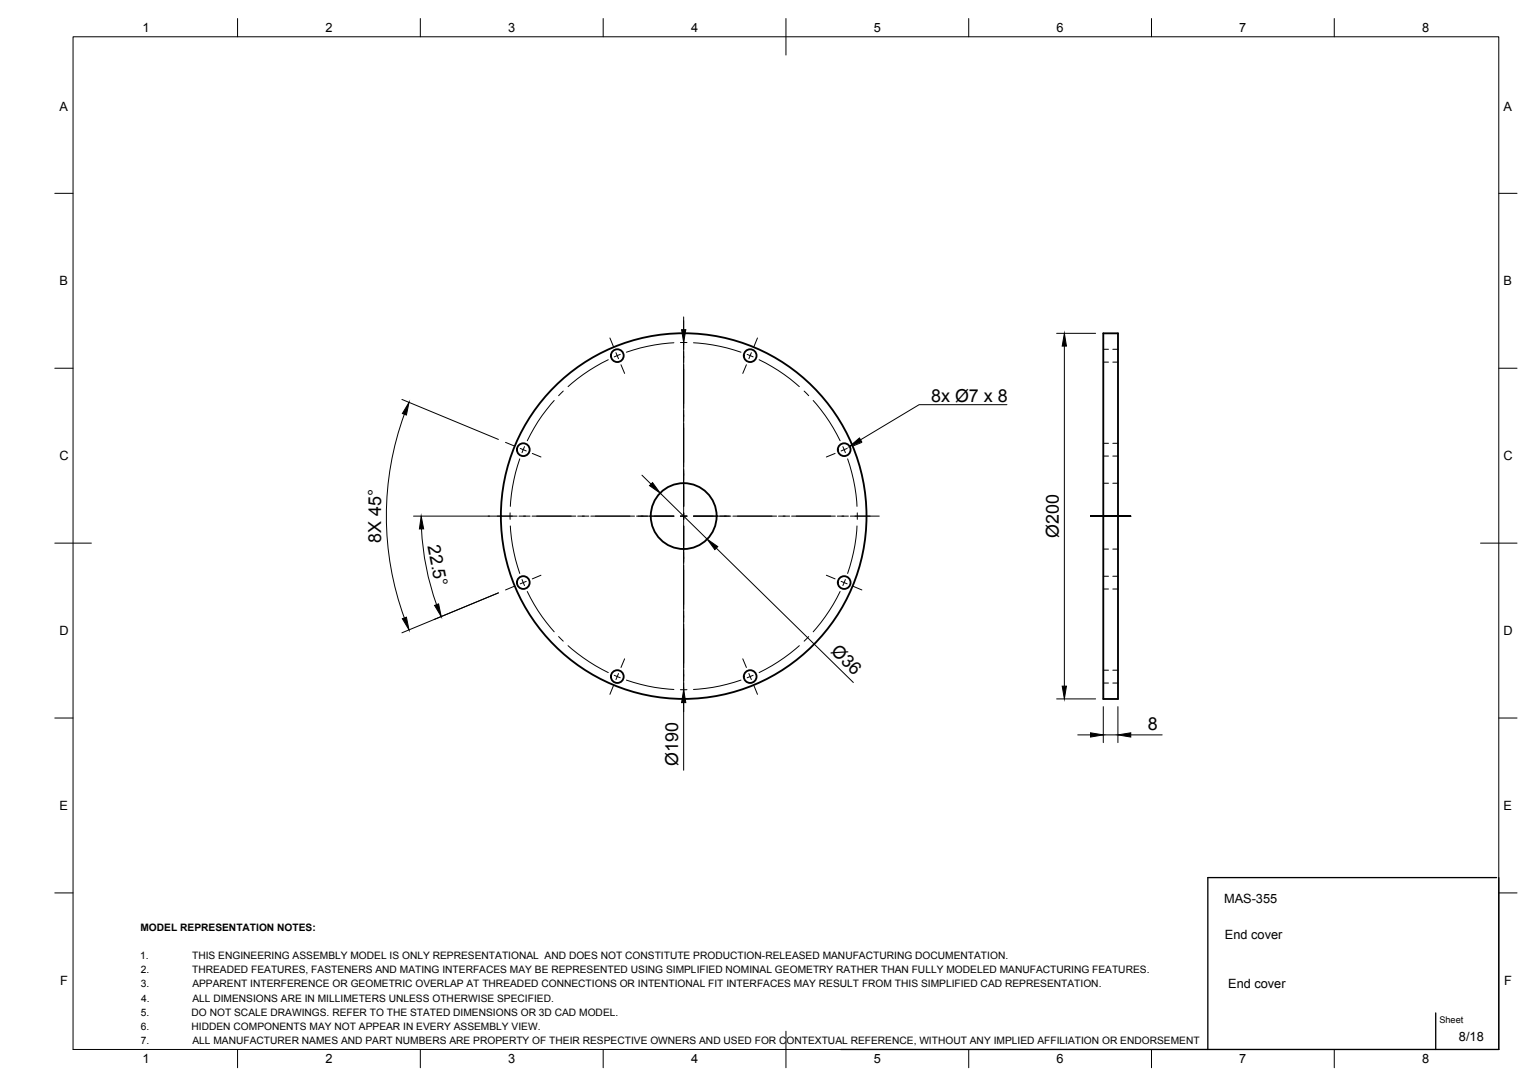
ISO-10303-21;
HEADER;
/* Generated by software containing ST-Developer
 * from STEP Tools, Inc. (www.steptools.com) 
 */

FILE_DESCRIPTION(
/* description */ ('Independent two-stage fixed-ring planetary gearbox,24/24/72 teeth,mod
ule2,20deg involutes,three planets per stage,4:1 x4:1=16:1. Native cut
-space/fillet/pattern tooth profiles derived from reusable gear blanks
; shared sun/planet/ring/carrier parts across both stages. Captured br
onze-journal input/carriers, headed retained planet pins, keyed inters
tage drive and modular keyed output interface. Native ideal gear links
; no torque, precision grade, production backlash/fits, lubrication, s
peed or life rating.'),
/* implementation_level */ '2;1');

FILE_NAME(
/* name */ 'End cover.step',
/* time_stamp */ '2026-11-08T19:10:00-08:00',
/* author */ (''),
/* organization */ (''),
/* preprocessor_version */ 'ST-DEVELOPER v20.2',
/* originating_system */ 'Autodesk Translation Framework v15.17.0.0',
/* authorisation */ '');

FILE_SCHEMA (('AUTOMOTIVE_DESIGN { 1 0 10303 214 3 1 1 }'));
ENDSEC;

DATA;
#10=MECHANICAL_DESIGN_GEOMETRIC_PRESENTATION_REPRESENTATION('',(#1165),#259224);
#1125=SHAPE_REPRESENTATION_RELATIONSHIP('SRR','None',#259372,#1145);
#1145=ADVANCED_BREP_SHAPE_REPRESENTATION('',(#1185),#259206);
#1165=STYLED_ITEM('',(#259481),#1185);
#1185=MANIFOLD_SOLID_BREP('Body1',#25152);
#1247=FACE_BOUND('',#3425,.T.);
#1248=FACE_BOUND('',#3426,.T.);
#1249=FACE_BOUND('',#3427,.T.);
#1250=FACE_BOUND('',#3428,.T.);
#1251=FACE_BOUND('',#3429,.T.);
#1252=FACE_BOUND('',#3430,.T.);
#1253=FACE_BOUND('',#3431,.T.);
#1254=FACE_BOUND('',#3432,.T.);
#1255=FACE_BOUND('',#3433,.T.);
#1256=FACE_BOUND('',#3435,.T.);
#1257=FACE_BOUND('',#3436,.T.);
#1258=FACE_BOUND('',#3437,.T.);
#1259=FACE_BOUND('',#3438,.T.);
#1260=FACE_BOUND('',#3439,.T.);
#1261=FACE_BOUND('',#3440,.T.);
#1262=FACE_BOUND('',#3441,.T.);
#1263=FACE_BOUND('',#3442,.T.);
#1264=FACE_BOUND('',#3443,.T.);
#1507=PLANE('',#25809);
#1508=PLANE('',#25810);
#2024=FACE_OUTER_BOUND('',#3414,.T.);
#2025=FACE_OUTER_BOUND('',#3415,.T.);
#2026=FACE_OUTER_BOUND('',#3416,.T.);
#2027=FACE_OUTER_BOUND('',#3417,.T.);
#2028=FACE_OUTER_BOUND('',#3418,.T.);
#2029=FACE_OUTER_BOUND('',#3419,.T.);
#2030=FACE_OUTER_BOUND('',#3420,.T.);
#2031=FACE_OUTER_BOUND('',#3421,.T.);
#2032=FACE_OUTER_BOUND('',#3422,.T.);
#2033=FACE_OUTER_BOUND('',#3423,.T.);
#2034=FACE_OUTER_BOUND('',#3424,.T.);
#2035=FACE_OUTER_BOUND('',#3434,.T.);
#3414=EDGE_LOOP('',(#17352,#17353,#17354,#17355));
#3415=EDGE_LOOP('',(#17356,#17357,#17358,#17359));
#3416=EDGE_LOOP('',(#17360,#17361,#17362,#17363));
#3417=EDGE_LOOP('',(#17364,#17365,#17366,#17367));
#3418=EDGE_LOOP('',(#17368,#17369,#17370,#17371));
#3419=EDGE_LOOP('',(#17372,#17373,#17374,#17375));
#3420=EDGE_LOOP('',(#17376,#17377,#17378,#17379));
#3421=EDGE_LOOP('',(#17380,#17381,#17382,#17383));
#3422=EDGE_LOOP('',(#17384,#17385,#17386,#17387));
#3423=EDGE_LOOP('',(#17388,#17389,#17390,#17391));
#3424=EDGE_LOOP('',(#17392));
#3425=EDGE_LOOP('',(#17393));
#3426=EDGE_LOOP('',(#17394));
#3427=EDGE_LOOP('',(#17395));
#3428=EDGE_LOOP('',(#17396));
#3429=EDGE_LOOP('',(#17397));
#3430=EDGE_LOOP('',(#17398));
#3431=EDGE_LOOP('',(#17399));
#3432=EDGE_LOOP('',(#17400));
#3433=EDGE_LOOP('',(#17401));
#3434=EDGE_LOOP('',(#17402));
#3435=EDGE_LOOP('',(#17403));
#3436=EDGE_LOOP('',(#17404));
#3437=EDGE_LOOP('',(#17405));
#3438=EDGE_LOOP('',(#17406));
#3439=EDGE_LOOP('',(#17407));
#3440=EDGE_LOOP('',(#17408));
#3441=EDGE_LOOP('',(#17409));
#3442=EDGE_LOOP('',(#17410));
#3443=EDGE_LOOP('',(#17411));
#4579=CIRCLE('',#25780,3.5);
#4580=CIRCLE('',#25781,3.5);
#4581=CIRCLE('',#25783,3.5);
#4582=CIRCLE('',#25784,3.5);
#4583=CIRCLE('',#25786,3.5);
#4584=CIRCLE('',#25787,3.5);
#4585=CIRCLE('',#25789,3.5);
#4586=CIRCLE('',#25790,3.5);
#4587=CIRCLE('',#25792,3.5);
#4588=CIRCLE('',#25793,3.5);
#4589=CIRCLE('',#25795,3.5);
#4590=CIRCLE('',#25796,3.5);
#4591=CIRCLE('',#25798,3.5);
#4592=CIRCLE('',#25799,3.5);
#4593=CIRCLE('',#25801,3.5);
#4594=CIRCLE('',#25802,3.5);
#4595=CIRCLE('',#25804,18.);
#4596=CIRCLE('',#25805,18.);
#4597=CIRCLE('',#25807,100.);
#4598=CIRCLE('',#25808,100.);
#6949=LINE('',#52233,#8134);
#6950=LINE('',#52239,#8135);
#6951=LINE('',#52245,#8136);
#6952=LINE('',#52251,#8137);
#6953=LINE('',#52257,#8138);
#6954=LINE('',#52263,#8139);
#6955=LINE('',#52269,#8140);
#6956=LINE('',#52275,#8141);
#6957=LINE('',#52281,#8142);
#6958=LINE('',#52287,#8143);
#8134=VECTOR('',#28396,3.5);
#8135=VECTOR('',#28403,3.5);
#8136=VECTOR('',#28410,3.5);
#8137=VECTOR('',#28417,3.5);
#8138=VECTOR('',#28424,3.5);
#8139=VECTOR('',#28431,3.5);
#8140=VECTOR('',#28438,3.5);
#8141=VECTOR('',#28445,3.5);
#8142=VECTOR('',#28452,18.);
#8143=VECTOR('',#28459,100.);
#9687=VERTEX_POINT('',#52230);
#9688=VERTEX_POINT('',#52232);
#9689=VERTEX_POINT('',#52236);
#9690=VERTEX_POINT('',#52238);
#9691=VERTEX_POINT('',#52242);
#9692=VERTEX_POINT('',#52244);
#9693=VERTEX_POINT('',#52248);
#9694=VERTEX_POINT('',#52250);
#9695=VERTEX_POINT('',#52254);
#9696=VERTEX_POINT('',#52256);
#9697=VERTEX_POINT('',#52260);
#9698=VERTEX_POINT('',#52262);
#9699=VERTEX_POINT('',#52266);
#9700=VERTEX_POINT('',#52268);
#9701=VERTEX_POINT('',#52272);
#9702=VERTEX_POINT('',#52274);
#9703=VERTEX_POINT('',#52278);
#9704=VERTEX_POINT('',#52280);
#9705=VERTEX_POINT('',#52284);
#9706=VERTEX_POINT('',#52286);
#12561=EDGE_CURVE('',#9687,#9687,#4579,.T.);
#12562=EDGE_CURVE('',#9687,#9688,#6949,.T.);
#12563=EDGE_CURVE('',#9688,#9688,#4580,.T.);
#12564=EDGE_CURVE('',#9689,#9689,#4581,.T.);
#12565=EDGE_CURVE('',#9689,#9690,#6950,.T.);
#12566=EDGE_CURVE('',#9690,#9690,#4582,.T.);
#12567=EDGE_CURVE('',#9691,#9691,#4583,.T.);
#12568=EDGE_CURVE('',#9691,#9692,#6951,.T.);
#12569=EDGE_CURVE('',#9692,#9692,#4584,.T.);
#12570=EDGE_CURVE('',#9693,#9693,#4585,.T.);
#12571=EDGE_CURVE('',#9693,#9694,#6952,.T.);
#12572=EDGE_CURVE('',#9694,#9694,#4586,.T.);
#12573=EDGE_CURVE('',#9695,#9695,#4587,.T.);
#12574=EDGE_CURVE('',#9695,#9696,#6953,.T.);
#12575=EDGE_CURVE('',#9696,#9696,#4588,.T.);
#12576=EDGE_CURVE('',#9697,#9697,#4589,.T.);
#12577=EDGE_CURVE('',#9697,#9698,#6954,.T.);
#12578=EDGE_CURVE('',#9698,#9698,#4590,.T.);
#12579=EDGE_CURVE('',#9699,#9699,#4591,.T.);
#12580=EDGE_CURVE('',#9699,#9700,#6955,.T.);
#12581=EDGE_CURVE('',#9700,#9700,#4592,.T.);
#12582=EDGE_CURVE('',#9701,#9701,#4593,.T.);
#12583=EDGE_CURVE('',#9701,#9702,#6956,.T.);
#12584=EDGE_CURVE('',#9702,#9702,#4594,.T.);
#12585=EDGE_CURVE('',#9703,#9703,#4595,.T.);
#12586=EDGE_CURVE('',#9703,#9704,#6957,.T.);
#12587=EDGE_CURVE('',#9704,#9704,#4596,.T.);
#12588=EDGE_CURVE('',#9705,#9705,#4597,.T.);
#12589=EDGE_CURVE('',#9705,#9706,#6958,.T.);
#12590=EDGE_CURVE('',#9706,#9706,#4598,.T.);
#17352=ORIENTED_EDGE('',*,*,#12561,.F.);
#17353=ORIENTED_EDGE('',*,*,#12562,.T.);
#17354=ORIENTED_EDGE('',*,*,#12563,.F.);
#17355=ORIENTED_EDGE('',*,*,#12562,.F.);
#17356=ORIENTED_EDGE('',*,*,#12564,.F.);
#17357=ORIENTED_EDGE('',*,*,#12565,.T.);
#17358=ORIENTED_EDGE('',*,*,#12566,.F.);
#17359=ORIENTED_EDGE('',*,*,#12565,.F.);
#17360=ORIENTED_EDGE('',*,*,#12567,.F.);
#17361=ORIENTED_EDGE('',*,*,#12568,.T.);
#17362=ORIENTED_EDGE('',*,*,#12569,.F.);
#17363=ORIENTED_EDGE('',*,*,#12568,.F.);
#17364=ORIENTED_EDGE('',*,*,#12570,.F.);
#17365=ORIENTED_EDGE('',*,*,#12571,.T.);
#17366=ORIENTED_EDGE('',*,*,#12572,.F.);
#17367=ORIENTED_EDGE('',*,*,#12571,.F.);
#17368=ORIENTED_EDGE('',*,*,#12573,.F.);
#17369=ORIENTED_EDGE('',*,*,#12574,.T.);
#17370=ORIENTED_EDGE('',*,*,#12575,.F.);
#17371=ORIENTED_EDGE('',*,*,#12574,.F.);
#17372=ORIENTED_EDGE('',*,*,#12576,.F.);
#17373=ORIENTED_EDGE('',*,*,#12577,.T.);
#17374=ORIENTED_EDGE('',*,*,#12578,.F.);
#17375=ORIENTED_EDGE('',*,*,#12577,.F.);
#17376=ORIENTED_EDGE('',*,*,#12579,.F.);
#17377=ORIENTED_EDGE('',*,*,#12580,.T.);
#17378=ORIENTED_EDGE('',*,*,#12581,.F.);
#17379=ORIENTED_EDGE('',*,*,#12580,.F.);
#17380=ORIENTED_EDGE('',*,*,#12582,.F.);
#17381=ORIENTED_EDGE('',*,*,#12583,.T.);
#17382=ORIENTED_EDGE('',*,*,#12584,.F.);
#17383=ORIENTED_EDGE('',*,*,#12583,.F.);
#17384=ORIENTED_EDGE('',*,*,#12585,.F.);
#17385=ORIENTED_EDGE('',*,*,#12586,.T.);
#17386=ORIENTED_EDGE('',*,*,#12587,.T.);
#17387=ORIENTED_EDGE('',*,*,#12586,.F.);
#17388=ORIENTED_EDGE('',*,*,#12588,.F.);
#17389=ORIENTED_EDGE('',*,*,#12589,.T.);
#17390=ORIENTED_EDGE('',*,*,#12590,.T.);
#17391=ORIENTED_EDGE('',*,*,#12589,.F.);
#17392=ORIENTED_EDGE('',*,*,#12588,.T.);
#17393=ORIENTED_EDGE('',*,*,#12585,.T.);
#17394=ORIENTED_EDGE('',*,*,#12582,.T.);
#17395=ORIENTED_EDGE('',*,*,#12579,.T.);
#17396=ORIENTED_EDGE('',*,*,#12576,.T.);
#17397=ORIENTED_EDGE('',*,*,#12573,.T.);
#17398=ORIENTED_EDGE('',*,*,#12570,.T.);
#17399=ORIENTED_EDGE('',*,*,#12567,.T.);
#17400=ORIENTED_EDGE('',*,*,#12564,.T.);
#17401=ORIENTED_EDGE('',*,*,#12561,.T.);
#17402=ORIENTED_EDGE('',*,*,#12590,.F.);
#17403=ORIENTED_EDGE('',*,*,#12587,.F.);
#17404=ORIENTED_EDGE('',*,*,#12584,.T.);
#17405=ORIENTED_EDGE('',*,*,#12581,.T.);
#17406=ORIENTED_EDGE('',*,*,#12578,.T.);
#17407=ORIENTED_EDGE('',*,*,#12575,.T.);
#17408=ORIENTED_EDGE('',*,*,#12572,.T.);
#17409=ORIENTED_EDGE('',*,*,#12569,.T.);
#17410=ORIENTED_EDGE('',*,*,#12566,.T.);
#17411=ORIENTED_EDGE('',*,*,#12563,.T.);
#23361=CYLINDRICAL_SURFACE('',#25779,3.5);
#23362=CYLINDRICAL_SURFACE('',#25782,3.5);
#23363=CYLINDRICAL_SURFACE('',#25785,3.5);
#23364=CYLINDRICAL_SURFACE('',#25788,3.5);
#23365=CYLINDRICAL_SURFACE('',#25791,3.5);
#23366=CYLINDRICAL_SURFACE('',#25794,3.5);
#23367=CYLINDRICAL_SURFACE('',#25797,3.5);
#23368=CYLINDRICAL_SURFACE('',#25800,3.5);
#23369=CYLINDRICAL_SURFACE('',#25803,18.);
#23370=CYLINDRICAL_SURFACE('',#25806,100.);
#24130=ADVANCED_FACE('',(#2024),#23361,.F.);
#24131=ADVANCED_FACE('',(#2025),#23362,.F.);
#24132=ADVANCED_FACE('',(#2026),#23363,.F.);
#24133=ADVANCED_FACE('',(#2027),#23364,.F.);
#24134=ADVANCED_FACE('',(#2028),#23365,.F.);
#24135=ADVANCED_FACE('',(#2029),#23366,.F.);
#24136=ADVANCED_FACE('',(#2030),#23367,.F.);
#24137=ADVANCED_FACE('',(#2031),#23368,.F.);
#24138=ADVANCED_FACE('',(#2032),#23369,.F.);
#24139=ADVANCED_FACE('',(#2033),#23370,.T.);
#24140=ADVANCED_FACE('',(#2034,#1247,#1248,#1249,#1250,#1251,#1252,#1253,
#1254,#1255),#1507,.T.);
#24141=ADVANCED_FACE('',(#2035,#1256,#1257,#1258,#1259,#1260,#1261,#1262,
#1263,#1264),#1508,.F.);
#25152=CLOSED_SHELL('',(#24130,#24131,#24132,#24133,#24134,#24135,#24136,
#24137,#24138,#24139,#24140,#24141));
#25778=AXIS2_PLACEMENT_3D('',#52228,#28390,#28391);
#25779=AXIS2_PLACEMENT_3D('',#52229,#28392,#28393);
#25780=AXIS2_PLACEMENT_3D('',#52231,#28394,#28395);
#25781=AXIS2_PLACEMENT_3D('',#52234,#28397,#28398);
#25782=AXIS2_PLACEMENT_3D('',#52235,#28399,#28400);
#25783=AXIS2_PLACEMENT_3D('',#52237,#28401,#28402);
#25784=AXIS2_PLACEMENT_3D('',#52240,#28404,#28405);
#25785=AXIS2_PLACEMENT_3D('',#52241,#28406,#28407);
#25786=AXIS2_PLACEMENT_3D('',#52243,#28408,#28409);
#25787=AXIS2_PLACEMENT_3D('',#52246,#28411,#28412);
#25788=AXIS2_PLACEMENT_3D('',#52247,#28413,#28414);
#25789=AXIS2_PLACEMENT_3D('',#52249,#28415,#28416);
#25790=AXIS2_PLACEMENT_3D('',#52252,#28418,#28419);
#25791=AXIS2_PLACEMENT_3D('',#52253,#28420,#28421);
#25792=AXIS2_PLACEMENT_3D('',#52255,#28422,#28423);
#25793=AXIS2_PLACEMENT_3D('',#52258,#28425,#28426);
#25794=AXIS2_PLACEMENT_3D('',#52259,#28427,#28428);
#25795=AXIS2_PLACEMENT_3D('',#52261,#28429,#28430);
#25796=AXIS2_PLACEMENT_3D('',#52264,#28432,#28433);
#25797=AXIS2_PLACEMENT_3D('',#52265,#28434,#28435);
#25798=AXIS2_PLACEMENT_3D('',#52267,#28436,#28437);
#25799=AXIS2_PLACEMENT_3D('',#52270,#28439,#28440);
#25800=AXIS2_PLACEMENT_3D('',#52271,#28441,#28442);
#25801=AXIS2_PLACEMENT_3D('',#52273,#28443,#28444);
#25802=AXIS2_PLACEMENT_3D('',#52276,#28446,#28447);
#25803=AXIS2_PLACEMENT_3D('',#52277,#28448,#28449);
#25804=AXIS2_PLACEMENT_3D('',#52279,#28450,#28451);
#25805=AXIS2_PLACEMENT_3D('',#52282,#28453,#28454);
#25806=AXIS2_PLACEMENT_3D('',#52283,#28455,#28456);
#25807=AXIS2_PLACEMENT_3D('',#52285,#28457,#28458);
#25808=AXIS2_PLACEMENT_3D('',#52288,#28460,#28461);
#25809=AXIS2_PLACEMENT_3D('',#52289,#28462,#28463);
#25810=AXIS2_PLACEMENT_3D('',#52290,#28464,#28465);
#28390=DIRECTION('axis',(0.,0.,1.));
#28391=DIRECTION('refdir',(1.,0.,0.));
#28392=DIRECTION('center_axis',(0.,0.,-1.));
#28393=DIRECTION('ref_axis',(1.,0.,0.));
#28394=DIRECTION('center_axis',(0.,0.,-1.));
#28395=DIRECTION('ref_axis',(1.,0.,0.));
#28396=DIRECTION('',(0.,0.,-1.));
#28397=DIRECTION('center_axis',(0.,0.,1.));
#28398=DIRECTION('ref_axis',(1.,0.,0.));
#28399=DIRECTION('center_axis',(0.,0.,-1.));
#28400=DIRECTION('ref_axis',(1.,0.,0.));
#28401=DIRECTION('center_axis',(0.,0.,-1.));
#28402=DIRECTION('ref_axis',(1.,0.,0.));
#28403=DIRECTION('',(0.,0.,-1.));
#28404=DIRECTION('center_axis',(0.,0.,1.));
#28405=DIRECTION('ref_axis',(1.,0.,0.));
#28406=DIRECTION('center_axis',(0.,0.,-1.));
#28407=DIRECTION('ref_axis',(1.,0.,0.));
#28408=DIRECTION('center_axis',(0.,0.,-1.));
#28409=DIRECTION('ref_axis',(1.,0.,0.));
#28410=DIRECTION('',(0.,0.,-1.));
#28411=DIRECTION('center_axis',(0.,0.,1.));
#28412=DIRECTION('ref_axis',(1.,0.,0.));
#28413=DIRECTION('center_axis',(0.,0.,-1.));
#28414=DIRECTION('ref_axis',(1.,0.,0.));
#28415=DIRECTION('center_axis',(0.,0.,-1.));
#28416=DIRECTION('ref_axis',(1.,0.,0.));
#28417=DIRECTION('',(0.,0.,-1.));
#28418=DIRECTION('center_axis',(0.,0.,1.));
#28419=DIRECTION('ref_axis',(1.,0.,0.));
#28420=DIRECTION('center_axis',(0.,0.,-1.));
#28421=DIRECTION('ref_axis',(1.,0.,0.));
#28422=DIRECTION('center_axis',(0.,0.,-1.));
#28423=DIRECTION('ref_axis',(1.,0.,0.));
#28424=DIRECTION('',(0.,0.,-1.));
#28425=DIRECTION('center_axis',(0.,0.,1.));
#28426=DIRECTION('ref_axis',(1.,0.,0.));
#28427=DIRECTION('center_axis',(0.,0.,-1.));
#28428=DIRECTION('ref_axis',(1.,0.,0.));
#28429=DIRECTION('center_axis',(0.,0.,-1.));
#28430=DIRECTION('ref_axis',(1.,0.,0.));
#28431=DIRECTION('',(0.,0.,-1.));
#28432=DIRECTION('center_axis',(0.,0.,1.));
#28433=DIRECTION('ref_axis',(1.,0.,0.));
#28434=DIRECTION('center_axis',(0.,0.,-1.));
#28435=DIRECTION('ref_axis',(1.,0.,0.));
#28436=DIRECTION('center_axis',(0.,0.,-1.));
#28437=DIRECTION('ref_axis',(1.,0.,0.));
#28438=DIRECTION('',(0.,0.,-1.));
#28439=DIRECTION('center_axis',(0.,0.,1.));
#28440=DIRECTION('ref_axis',(1.,0.,0.));
#28441=DIRECTION('center_axis',(0.,0.,-1.));
#28442=DIRECTION('ref_axis',(1.,0.,0.));
#28443=DIRECTION('center_axis',(0.,0.,-1.));
#28444=DIRECTION('ref_axis',(1.,0.,0.));
#28445=DIRECTION('',(0.,0.,-1.));
#28446=DIRECTION('center_axis',(0.,0.,1.));
#28447=DIRECTION('ref_axis',(1.,0.,0.));
#28448=DIRECTION('center_axis',(0.,0.,1.));
#28449=DIRECTION('ref_axis',(1.,0.,0.));
#28450=DIRECTION('center_axis',(0.,0.,-1.));
#28451=DIRECTION('ref_axis',(1.,0.,0.));
#28452=DIRECTION('',(0.,0.,-1.));
#28453=DIRECTION('center_axis',(0.,0.,-1.));
#28454=DIRECTION('ref_axis',(1.,0.,0.));
#28455=DIRECTION('center_axis',(0.,0.,1.));
#28456=DIRECTION('ref_axis',(1.,0.,0.));
#28457=DIRECTION('center_axis',(0.,0.,1.));
#28458=DIRECTION('ref_axis',(1.,0.,0.));
#28459=DIRECTION('',(0.,0.,-1.));
#28460=DIRECTION('center_axis',(0.,0.,1.));
#28461=DIRECTION('ref_axis',(1.,0.,0.));
#28462=DIRECTION('center_axis',(0.,0.,1.));
#28463=DIRECTION('ref_axis',(1.,0.,0.));
#28464=DIRECTION('center_axis',(0.,0.,1.));
#28465=DIRECTION('ref_axis',(1.,0.,0.));
#52228=CARTESIAN_POINT('',(0.,0.,0.));
#52229=CARTESIAN_POINT('Origin',(36.3549260746835,-87.7685555885722,4.));
#52230=CARTESIAN_POINT('',(32.8549260746835,-87.7685555885722,8.));
#52231=CARTESIAN_POINT('Origin',(36.3549260746835,-87.7685555885722,8.));
#52232=CARTESIAN_POINT('',(32.8549260746835,-87.7685555885722,0.));
#52233=CARTESIAN_POINT('',(32.8549260746835,-87.7685555885722,4.));
#52234=CARTESIAN_POINT('Origin',(36.3549260746835,-87.7685555885722,0.));
#52235=CARTESIAN_POINT('Origin',(-87.7685555885722,-36.3549260746835,4.));
#52236=CARTESIAN_POINT('',(-91.2685555885722,-36.3549260746835,8.));
#52237=CARTESIAN_POINT('Origin',(-87.7685555885722,-36.3549260746835,8.));
#52238=CARTESIAN_POINT('',(-91.2685555885722,-36.3549260746835,0.));
#52239=CARTESIAN_POINT('',(-91.2685555885722,-36.3549260746835,4.));
#52240=CARTESIAN_POINT('Origin',(-87.7685555885722,-36.3549260746835,0.));
#52241=CARTESIAN_POINT('Origin',(-36.3549260746835,87.7685555885722,4.));
#52242=CARTESIAN_POINT('',(-39.8549260746835,87.7685555885722,8.));
#52243=CARTESIAN_POINT('Origin',(-36.3549260746835,87.7685555885722,8.));
#52244=CARTESIAN_POINT('',(-39.8549260746835,87.7685555885722,0.));
#52245=CARTESIAN_POINT('',(-39.8549260746835,87.7685555885722,4.));
#52246=CARTESIAN_POINT('Origin',(-36.3549260746835,87.7685555885722,0.));
#52247=CARTESIAN_POINT('Origin',(87.7685555885722,36.3549260746835,4.));
#52248=CARTESIAN_POINT('',(84.2685555885723,36.3549260746835,8.));
#52249=CARTESIAN_POINT('Origin',(87.7685555885722,36.3549260746835,8.));
#52250=CARTESIAN_POINT('',(84.2685555885723,36.3549260746835,0.));
#52251=CARTESIAN_POINT('',(84.2685555885723,36.3549260746835,4.));
#52252=CARTESIAN_POINT('Origin',(87.7685555885722,36.3549260746835,0.));
#52253=CARTESIAN_POINT('Origin',(36.3549260746835,87.7685555885722,4.));
#52254=CARTESIAN_POINT('',(32.8549260746835,87.7685555885722,8.));
#52255=CARTESIAN_POINT('Origin',(36.3549260746835,87.7685555885722,8.));
#52256=CARTESIAN_POINT('',(32.8549260746835,87.7685555885722,0.));
#52257=CARTESIAN_POINT('',(32.8549260746835,87.7685555885722,4.));
#52258=CARTESIAN_POINT('Origin',(36.3549260746835,87.7685555885722,0.));
#52259=CARTESIAN_POINT('Origin',(-87.7685555885722,36.3549260746835,4.));
#52260=CARTESIAN_POINT('',(-91.2685555885722,36.3549260746835,8.));
#52261=CARTESIAN_POINT('Origin',(-87.7685555885722,36.3549260746835,8.));
#52262=CARTESIAN_POINT('',(-91.2685555885722,36.3549260746835,0.));
#52263=CARTESIAN_POINT('',(-91.2685555885722,36.3549260746835,4.));
#52264=CARTESIAN_POINT('Origin',(-87.7685555885722,36.3549260746835,0.));
#52265=CARTESIAN_POINT('Origin',(-36.3549260746835,-87.7685555885722,4.));
#52266=CARTESIAN_POINT('',(-39.8549260746835,-87.7685555885722,8.));
#52267=CARTESIAN_POINT('Origin',(-36.3549260746835,-87.7685555885722,8.));
#52268=CARTESIAN_POINT('',(-39.8549260746835,-87.7685555885722,0.));
#52269=CARTESIAN_POINT('',(-39.8549260746835,-87.7685555885722,4.));
#52270=CARTESIAN_POINT('Origin',(-36.3549260746835,-87.7685555885722,0.));
#52271=CARTESIAN_POINT('Origin',(87.7685555885722,-36.3549260746835,4.));
#52272=CARTESIAN_POINT('',(84.2685555885723,-36.3549260746835,8.));
#52273=CARTESIAN_POINT('Origin',(87.7685555885722,-36.3549260746835,8.));
#52274=CARTESIAN_POINT('',(84.2685555885723,-36.3549260746835,0.));
#52275=CARTESIAN_POINT('',(84.2685555885723,-36.3549260746835,4.));
#52276=CARTESIAN_POINT('Origin',(87.7685555885722,-36.3549260746835,0.));
#52277=CARTESIAN_POINT('Origin',(0.,0.,0.));
#52278=CARTESIAN_POINT('',(-18.,-2.20436423846524E-15,8.));
#52279=CARTESIAN_POINT('Origin',(0.,0.,8.));
#52280=CARTESIAN_POINT('',(-18.,-2.20436423846524E-15,0.));
#52281=CARTESIAN_POINT('',(-18.,-2.20436423846524E-15,0.));
#52282=CARTESIAN_POINT('Origin',(0.,0.,0.));
#52283=CARTESIAN_POINT('Origin',(0.,0.,0.));
#52284=CARTESIAN_POINT('',(-100.,-1.22464679914735E-14,8.));
#52285=CARTESIAN_POINT('Origin',(0.,0.,8.));
#52286=CARTESIAN_POINT('',(-100.,-1.22464679914735E-14,0.));
#52287=CARTESIAN_POINT('',(-100.,-1.22464679914735E-14,0.));
#52288=CARTESIAN_POINT('Origin',(0.,0.,0.));
#52289=CARTESIAN_POINT('Origin',(0.,0.,8.));
#52290=CARTESIAN_POINT('Origin',(0.,0.,0.));
#259184=UNCERTAINTY_MEASURE_WITH_UNIT(LENGTH_MEASURE(0.01),#259225,
'DISTANCE_ACCURACY_VALUE',
'Maximum model space distance between geometric entities at asserted c
onnectivities');
#259202=UNCERTAINTY_MEASURE_WITH_UNIT(LENGTH_MEASURE(0.01),#259225,
'DISTANCE_ACCURACY_VALUE',
'Maximum model space distance between geometric entities at asserted c
onnectivities');
#259206=(
GEOMETRIC_REPRESENTATION_CONTEXT(3)
GLOBAL_UNCERTAINTY_ASSIGNED_CONTEXT((#259184))
GLOBAL_UNIT_ASSIGNED_CONTEXT((#259225,#259227,#259228))
REPRESENTATION_CONTEXT('','3D')
);
#259224=(
GEOMETRIC_REPRESENTATION_CONTEXT(3)
GLOBAL_UNCERTAINTY_ASSIGNED_CONTEXT((#259202))
GLOBAL_UNIT_ASSIGNED_CONTEXT((#259225,#259227,#259228))
REPRESENTATION_CONTEXT('','3D')
);
#259225=(
LENGTH_UNIT()
NAMED_UNIT(*)
SI_UNIT(.MILLI.,.METRE.)
);
#259227=(
NAMED_UNIT(*)
PLANE_ANGLE_UNIT()
SI_UNIT($,.RADIAN.)
);
#259228=(
NAMED_UNIT(*)
SI_UNIT($,.STERADIAN.)
SOLID_ANGLE_UNIT()
);
#259232=SHAPE_DEFINITION_REPRESENTATION(#259253,#259372);
#259253=PRODUCT_DEFINITION_SHAPE('',$,#259394);
#259372=SHAPE_REPRESENTATION('',(#25778),#259206);
#259390=PRODUCT_DEFINITION_CONTEXT('part definition',#259455,'design');
#259394=PRODUCT_DEFINITION('End cover','End cover',#259415,#259390);
#259415=PRODUCT_DEFINITION_FORMATION('',$,#259460);
#259455=APPLICATION_CONTEXT(
'Core Data for Automotive Mechanical Design Process');
#259456=PRODUCT_CONTEXT('part definition',#259455,'mechanical');
#259460=PRODUCT('End cover','End cover',$,(#259456));
#259481=PRESENTATION_STYLE_ASSIGNMENT((#259496));
#259496=SURFACE_STYLE_USAGE(.BOTH.,#259511);
#259511=SURFACE_SIDE_STYLE('',(#259526));
#259526=SURFACE_STYLE_FILL_AREA(#259541);
#259541=FILL_AREA_STYLE('Cover sky blue',(#259556));
#259556=FILL_AREA_STYLE_COLOUR('Cover sky blue',#259571);
#259571=COLOUR_RGB('Cover sky blue',0.317647058823529,0.686274509803922,
0.890196078431372);
ENDSEC;
END-ISO-10303-21;
